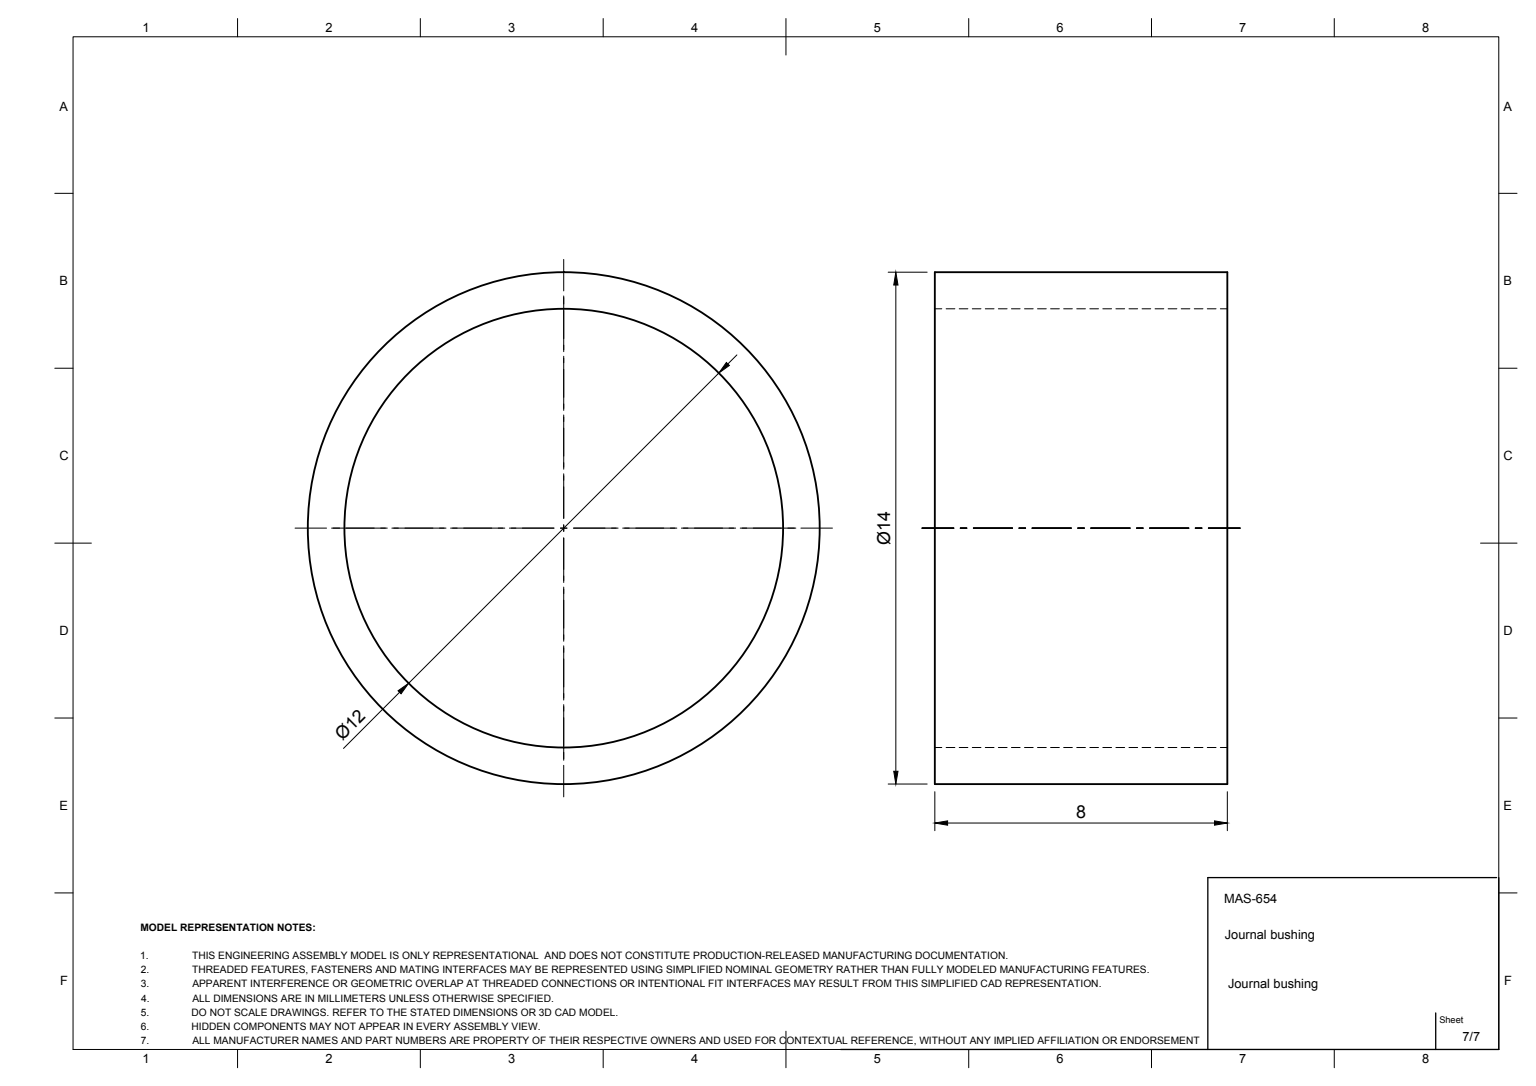
ISO-10303-21;
HEADER;
/* Generated by software containing ST-Developer
 * from STEP Tools, Inc. (www.steptools.com) 
 */

FILE_DESCRIPTION(
/* description */ ('Independent four-jaw lathe chuck,200mm body,40mm bore,36\X2\2013\X0\7
6mm nominal opposed jaw opening. Four shared machined T-jaws and model
ed partial M12x1.75 feed screws, native independent screw/slider links
, removable bolted bronze-bearing cartridges, fully captured ring/wash
er/head thrust stacks and registered bolted backplate. Custom spindle 
interface; no compatibility, speed, grip force or safety rating assign
ed.'),
/* implementation_level */ '2;1');

FILE_NAME(
/* name */ 'Journal bushing.step',
/* time_stamp */ '2026-11-09T20:24:54-08:00',
/* author */ (''),
/* organization */ (''),
/* preprocessor_version */ 'ST-DEVELOPER v20.2',
/* originating_system */ 'Autodesk Translation Framework v15.17.0.0',
/* authorisation */ '');

FILE_SCHEMA (('AUTOMOTIVE_DESIGN { 1 0 10303 214 3 1 1 }'));
ENDSEC;

DATA;
#10=MECHANICAL_DESIGN_GEOMETRIC_PRESENTATION_REPRESENTATION('',(#242),#69491);
#220=SHAPE_REPRESENTATION_RELATIONSHIP('SRR','None',#69577,#231);
#231=ADVANCED_BREP_SHAPE_REPRESENTATION('',(#253),#69486);
#242=STYLED_ITEM('',(#69641),#253);
#253=MANIFOLD_SOLID_BREP('Body1',#14737);
#355=FACE_BOUND('',#1957,.T.);
#356=FACE_BOUND('',#1959,.T.);
#496=PLANE('',#15604);
#497=PLANE('',#15605);
#1116=FACE_OUTER_BOUND('',#1954,.T.);
#1117=FACE_OUTER_BOUND('',#1955,.T.);
#1118=FACE_OUTER_BOUND('',#1956,.T.);
#1119=FACE_OUTER_BOUND('',#1958,.T.);
#1954=EDGE_LOOP('',(#12335,#12336,#12337,#12338));
#1955=EDGE_LOOP('',(#12339,#12340,#12341,#12342));
#1956=EDGE_LOOP('',(#12343));
#1957=EDGE_LOOP('',(#12344));
#1958=EDGE_LOOP('',(#12345));
#1959=EDGE_LOOP('',(#12346));
#2319=CIRCLE('',#15599,6.);
#2320=CIRCLE('',#15600,6.);
#2321=CIRCLE('',#15602,7.);
#2322=CIRCLE('',#15603,7.);
#4186=LINE('',#59267,#5034);
#4187=LINE('',#59273,#5035);
#5034=VECTOR('',#17994,6.);
#5035=VECTOR('',#18001,7.);
#6353=VERTEX_POINT('',#59264);
#6354=VERTEX_POINT('',#59266);
#6355=VERTEX_POINT('',#59270);
#6356=VERTEX_POINT('',#59272);
#8404=EDGE_CURVE('',#6353,#6353,#2319,.T.);
#8405=EDGE_CURVE('',#6353,#6354,#4186,.T.);
#8406=EDGE_CURVE('',#6354,#6354,#2320,.T.);
#8407=EDGE_CURVE('',#6355,#6355,#2321,.T.);
#8408=EDGE_CURVE('',#6355,#6356,#4187,.T.);
#8409=EDGE_CURVE('',#6356,#6356,#2322,.T.);
#12335=ORIENTED_EDGE('',*,*,#8404,.F.);
#12336=ORIENTED_EDGE('',*,*,#8405,.T.);
#12337=ORIENTED_EDGE('',*,*,#8406,.T.);
#12338=ORIENTED_EDGE('',*,*,#8405,.F.);
#12339=ORIENTED_EDGE('',*,*,#8407,.F.);
#12340=ORIENTED_EDGE('',*,*,#8408,.T.);
#12341=ORIENTED_EDGE('',*,*,#8409,.T.);
#12342=ORIENTED_EDGE('',*,*,#8408,.F.);
#12343=ORIENTED_EDGE('',*,*,#8407,.T.);
#12344=ORIENTED_EDGE('',*,*,#8404,.T.);
#12345=ORIENTED_EDGE('',*,*,#8409,.F.);
#12346=ORIENTED_EDGE('',*,*,#8406,.F.);
#13796=CYLINDRICAL_SURFACE('',#15598,6.);
#13797=CYLINDRICAL_SURFACE('',#15601,7.);
#14544=ADVANCED_FACE('',(#1116),#13796,.F.);
#14545=ADVANCED_FACE('',(#1117),#13797,.T.);
#14546=ADVANCED_FACE('',(#1118,#355),#496,.T.);
#14547=ADVANCED_FACE('',(#1119,#356),#497,.F.);
#14737=CLOSED_SHELL('',(#14544,#14545,#14546,#14547));
#15597=AXIS2_PLACEMENT_3D('',#59262,#17988,#17989);
#15598=AXIS2_PLACEMENT_3D('',#59263,#17990,#17991);
#15599=AXIS2_PLACEMENT_3D('',#59265,#17992,#17993);
#15600=AXIS2_PLACEMENT_3D('',#59268,#17995,#17996);
#15601=AXIS2_PLACEMENT_3D('',#59269,#17997,#17998);
#15602=AXIS2_PLACEMENT_3D('',#59271,#17999,#18000);
#15603=AXIS2_PLACEMENT_3D('',#59274,#18002,#18003);
#15604=AXIS2_PLACEMENT_3D('',#59275,#18004,#18005);
#15605=AXIS2_PLACEMENT_3D('',#59276,#18006,#18007);
#17988=DIRECTION('axis',(0.,0.,1.));
#17989=DIRECTION('refdir',(1.,0.,0.));
#17990=DIRECTION('center_axis',(0.,0.,1.));
#17991=DIRECTION('ref_axis',(1.,0.,0.));
#17992=DIRECTION('center_axis',(0.,0.,-1.));
#17993=DIRECTION('ref_axis',(1.,0.,0.));
#17994=DIRECTION('',(0.,0.,-1.));
#17995=DIRECTION('center_axis',(0.,0.,-1.));
#17996=DIRECTION('ref_axis',(1.,0.,0.));
#17997=DIRECTION('center_axis',(0.,0.,1.));
#17998=DIRECTION('ref_axis',(1.,0.,0.));
#17999=DIRECTION('center_axis',(0.,0.,1.));
#18000=DIRECTION('ref_axis',(1.,0.,0.));
#18001=DIRECTION('',(0.,0.,-1.));
#18002=DIRECTION('center_axis',(0.,0.,1.));
#18003=DIRECTION('ref_axis',(1.,0.,0.));
#18004=DIRECTION('center_axis',(0.,0.,1.));
#18005=DIRECTION('ref_axis',(1.,0.,0.));
#18006=DIRECTION('center_axis',(0.,0.,1.));
#18007=DIRECTION('ref_axis',(1.,0.,0.));
#59262=CARTESIAN_POINT('',(0.,0.,0.));
#59263=CARTESIAN_POINT('Origin',(0.,0.,0.));
#59264=CARTESIAN_POINT('',(-6.,-7.34788079488412E-16,8.));
#59265=CARTESIAN_POINT('Origin',(0.,0.,8.));
#59266=CARTESIAN_POINT('',(-6.,-7.34788079488412E-16,0.));
#59267=CARTESIAN_POINT('',(-6.,-7.34788079488412E-16,0.));
#59268=CARTESIAN_POINT('Origin',(0.,0.,0.));
#59269=CARTESIAN_POINT('Origin',(0.,0.,0.));
#59270=CARTESIAN_POINT('',(-7.,-8.57252759403147E-16,8.));
#59271=CARTESIAN_POINT('Origin',(0.,0.,8.));
#59272=CARTESIAN_POINT('',(-7.,-8.57252759403147E-16,0.));
#59273=CARTESIAN_POINT('',(-7.,-8.57252759403147E-16,0.));
#59274=CARTESIAN_POINT('Origin',(0.,0.,0.));
#59275=CARTESIAN_POINT('Origin',(0.,0.,8.));
#59276=CARTESIAN_POINT('Origin',(0.,0.,0.));
#69473=UNCERTAINTY_MEASURE_WITH_UNIT(LENGTH_MEASURE(0.01),#69492,
'DISTANCE_ACCURACY_VALUE',
'Maximum model space distance between geometric entities at asserted c
onnectivities');
#69478=UNCERTAINTY_MEASURE_WITH_UNIT(LENGTH_MEASURE(0.01),#69492,
'DISTANCE_ACCURACY_VALUE',
'Maximum model space distance between geometric entities at asserted c
onnectivities');
#69486=(
GEOMETRIC_REPRESENTATION_CONTEXT(3)
GLOBAL_UNCERTAINTY_ASSIGNED_CONTEXT((#69473))
GLOBAL_UNIT_ASSIGNED_CONTEXT((#69492,#69494,#69495))
REPRESENTATION_CONTEXT('','3D')
);
#69491=(
GEOMETRIC_REPRESENTATION_CONTEXT(3)
GLOBAL_UNCERTAINTY_ASSIGNED_CONTEXT((#69478))
GLOBAL_UNIT_ASSIGNED_CONTEXT((#69492,#69494,#69495))
REPRESENTATION_CONTEXT('','3D')
);
#69492=(
LENGTH_UNIT()
NAMED_UNIT(*)
SI_UNIT(.MILLI.,.METRE.)
);
#69494=(
NAMED_UNIT(*)
PLANE_ANGLE_UNIT()
SI_UNIT($,.RADIAN.)
);
#69495=(
NAMED_UNIT(*)
SI_UNIT($,.STERADIAN.)
SOLID_ANGLE_UNIT()
);
#69503=SHAPE_DEFINITION_REPRESENTATION(#69515,#69577);
#69515=PRODUCT_DEFINITION_SHAPE('',$,#69590);
#69577=SHAPE_REPRESENTATION('',(#15597),#69486);
#69582=PRODUCT_DEFINITION_CONTEXT('part definition',#69620,'design');
#69590=PRODUCT_DEFINITION('Journal bushing','Journal bushing',#69602,#69582);
#69602=PRODUCT_DEFINITION_FORMATION('',$,#69629);
#69620=APPLICATION_CONTEXT(
'Core Data for Automotive Mechanical Design Process');
#69621=PRODUCT_CONTEXT('part definition',#69620,'mechanical');
#69629=PRODUCT('Journal bushing','Journal bushing',$,(#69621));
#69641=PRESENTATION_STYLE_ASSIGNMENT((#69651));
#69651=SURFACE_STYLE_USAGE(.BOTH.,#69661);
#69661=SURFACE_SIDE_STYLE('',(#69671));
#69671=SURFACE_STYLE_FILL_AREA(#69681);
#69681=FILL_AREA_STYLE('Bearing light gray',(#69691));
#69691=FILL_AREA_STYLE_COLOUR('Bearing light gray',#69701);
#69701=COLOUR_RGB('Bearing light gray',0.725490196078431,0.752941176470588,
0.792156862745098);
ENDSEC;
END-ISO-10303-21;
